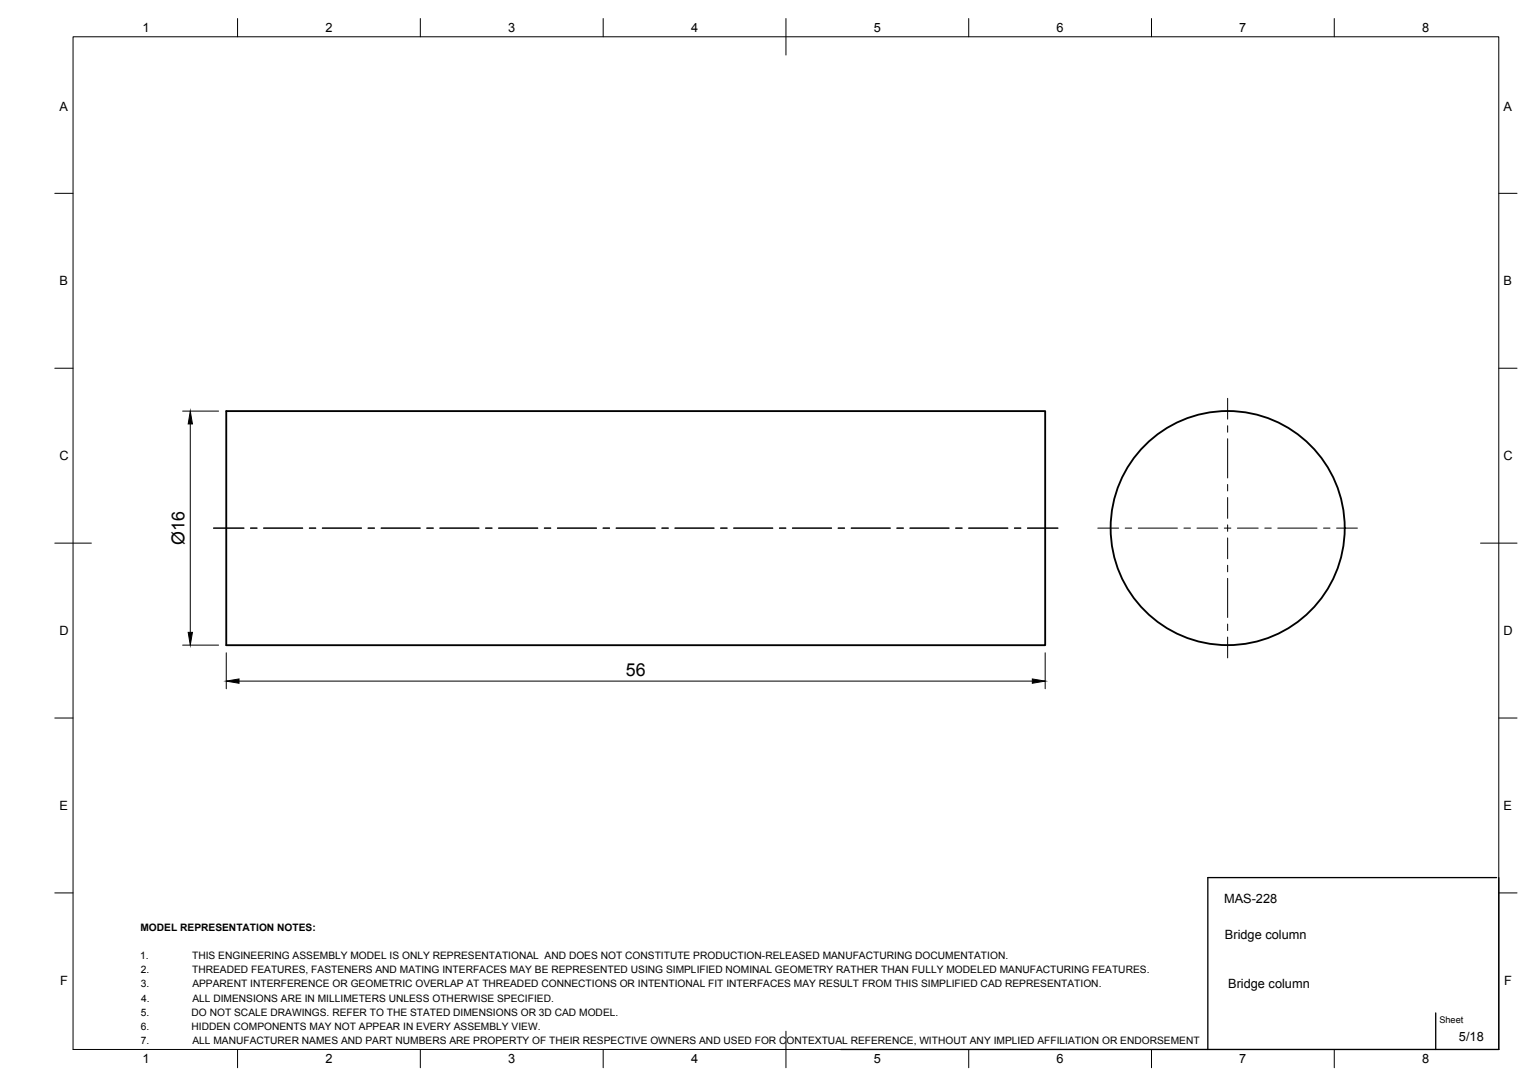
ISO-10303-21;
HEADER;
/* Generated by software containing ST-Developer
 * from STEP Tools, Inc. (www.steptools.com) 
 */

FILE_DESCRIPTION(
/* description */ ('Independent Peaucellier-Lipkin straight-line linkage. Radius arms 100
 mm, inversion-cell links 60 mm, crank radius and fixed-pivot spacing 
32 mm. Inversion constant 6400 mm squared, nominal output straight lin
e X=100 mm. Overhead bearing bridge clears the layered moving links. N
o accuracy or load rating assigned.'),
/* implementation_level */ '2;1');

FILE_NAME(
/* name */ 'Bridge column.step',
/* time_stamp */ '2026-11-09T18:06:16-08:00',
/* author */ (''),
/* organization */ (''),
/* preprocessor_version */ 'ST-DEVELOPER v20.2',
/* originating_system */ 'Autodesk Translation Framework v15.17.0.0',
/* authorisation */ '');

FILE_SCHEMA (('AUTOMOTIVE_DESIGN { 1 0 10303 214 3 1 1 }'));
ENDSEC;

DATA;
#10=MECHANICAL_DESIGN_GEOMETRIC_PRESENTATION_REPRESENTATION('',(#286),#3581);
#252=SHAPE_REPRESENTATION_RELATIONSHIP('SRR','None',#3686,#269);
#269=ADVANCED_BREP_SHAPE_REPRESENTATION('',(#303),#3568);
#286=STYLED_ITEM('',(#3777),#303);
#303=MANIFOLD_SOLID_BREP('Body1',#1872);
#382=PLANE('',#2136);
#383=PLANE('',#2137);
#455=FACE_OUTER_BOUND('',#584,.T.);
#456=FACE_OUTER_BOUND('',#585,.T.);
#457=FACE_OUTER_BOUND('',#586,.T.);
#584=EDGE_LOOP('',(#1448,#1449,#1450,#1451));
#585=EDGE_LOOP('',(#1452));
#586=EDGE_LOOP('',(#1453));
#737=LINE('',#3179,#835);
#835=VECTOR('',#2525,8.);
#915=CIRCLE('',#2134,8.);
#916=CIRCLE('',#2135,8.);
#1033=VERTEX_POINT('',#3176);
#1034=VERTEX_POINT('',#3178);
#1186=EDGE_CURVE('',#1033,#1033,#915,.T.);
#1187=EDGE_CURVE('',#1033,#1034,#737,.T.);
#1188=EDGE_CURVE('',#1034,#1034,#916,.T.);
#1448=ORIENTED_EDGE('',*,*,#1186,.F.);
#1449=ORIENTED_EDGE('',*,*,#1187,.T.);
#1450=ORIENTED_EDGE('',*,*,#1188,.T.);
#1451=ORIENTED_EDGE('',*,*,#1187,.F.);
#1452=ORIENTED_EDGE('',*,*,#1186,.T.);
#1453=ORIENTED_EDGE('',*,*,#1188,.F.);
#1720=CYLINDRICAL_SURFACE('',#2133,8.);
#1787=ADVANCED_FACE('',(#455),#1720,.T.);
#1788=ADVANCED_FACE('',(#456),#382,.T.);
#1789=ADVANCED_FACE('',(#457),#383,.F.);
#1872=CLOSED_SHELL('',(#1787,#1788,#1789));
#2132=AXIS2_PLACEMENT_3D('',#3174,#2519,#2520);
#2133=AXIS2_PLACEMENT_3D('',#3175,#2521,#2522);
#2134=AXIS2_PLACEMENT_3D('',#3177,#2523,#2524);
#2135=AXIS2_PLACEMENT_3D('',#3180,#2526,#2527);
#2136=AXIS2_PLACEMENT_3D('',#3181,#2528,#2529);
#2137=AXIS2_PLACEMENT_3D('',#3182,#2530,#2531);
#2519=DIRECTION('axis',(0.,0.,1.));
#2520=DIRECTION('refdir',(1.,0.,0.));
#2521=DIRECTION('center_axis',(0.,0.,1.));
#2522=DIRECTION('ref_axis',(1.,0.,0.));
#2523=DIRECTION('center_axis',(0.,0.,1.));
#2524=DIRECTION('ref_axis',(1.,0.,0.));
#2525=DIRECTION('',(0.,0.,-1.));
#2526=DIRECTION('center_axis',(0.,0.,1.));
#2527=DIRECTION('ref_axis',(1.,0.,0.));
#2528=DIRECTION('center_axis',(0.,0.,1.));
#2529=DIRECTION('ref_axis',(1.,0.,0.));
#2530=DIRECTION('center_axis',(0.,0.,1.));
#2531=DIRECTION('ref_axis',(1.,0.,0.));
#3174=CARTESIAN_POINT('',(0.,0.,0.));
#3175=CARTESIAN_POINT('Origin',(0.,0.,0.));
#3176=CARTESIAN_POINT('',(-8.,-9.79717439317883E-16,56.));
#3177=CARTESIAN_POINT('Origin',(0.,0.,56.));
#3178=CARTESIAN_POINT('',(-8.,-9.79717439317883E-16,0.));
#3179=CARTESIAN_POINT('',(-8.,-9.79717439317883E-16,0.));
#3180=CARTESIAN_POINT('Origin',(0.,0.,0.));
#3181=CARTESIAN_POINT('Origin',(0.,0.,56.));
#3182=CARTESIAN_POINT('Origin',(0.,0.,0.));
#3549=UNCERTAINTY_MEASURE_WITH_UNIT(LENGTH_MEASURE(0.01),#3582,
'DISTANCE_ACCURACY_VALUE',
'Maximum model space distance between geometric entities at asserted c
onnectivities');
#3562=UNCERTAINTY_MEASURE_WITH_UNIT(LENGTH_MEASURE(0.01),#3582,
'DISTANCE_ACCURACY_VALUE',
'Maximum model space distance between geometric entities at asserted c
onnectivities');
#3568=(
GEOMETRIC_REPRESENTATION_CONTEXT(3)
GLOBAL_UNCERTAINTY_ASSIGNED_CONTEXT((#3549))
GLOBAL_UNIT_ASSIGNED_CONTEXT((#3582,#3584,#3585))
REPRESENTATION_CONTEXT('','3D')
);
#3581=(
GEOMETRIC_REPRESENTATION_CONTEXT(3)
GLOBAL_UNCERTAINTY_ASSIGNED_CONTEXT((#3562))
GLOBAL_UNIT_ASSIGNED_CONTEXT((#3582,#3584,#3585))
REPRESENTATION_CONTEXT('','3D')
);
#3582=(
LENGTH_UNIT()
NAMED_UNIT(*)
SI_UNIT(.MILLI.,.METRE.)
);
#3584=(
NAMED_UNIT(*)
PLANE_ANGLE_UNIT()
SI_UNIT($,.RADIAN.)
);
#3585=(
NAMED_UNIT(*)
SI_UNIT($,.STERADIAN.)
SOLID_ANGLE_UNIT()
);
#3591=SHAPE_DEFINITION_REPRESENTATION(#3609,#3686);
#3609=PRODUCT_DEFINITION_SHAPE('',$,#3705);
#3686=SHAPE_REPRESENTATION('',(#2132),#3568);
#3699=PRODUCT_DEFINITION_CONTEXT('part definition',#3755,'design');
#3705=PRODUCT_DEFINITION('Bridge column','Bridge column',#3723,#3699);
#3723=PRODUCT_DEFINITION_FORMATION('',$,#3762);
#3755=APPLICATION_CONTEXT(
'Core Data for Automotive Mechanical Design Process');
#3756=PRODUCT_CONTEXT('part definition',#3755,'mechanical');
#3762=PRODUCT('Bridge column','Bridge column',$,(#3756));
#3777=PRESENTATION_STYLE_ASSIGNMENT((#3790));
#3790=SURFACE_STYLE_USAGE(.BOTH.,#3803);
#3803=SURFACE_SIDE_STYLE('',(#3816));
#3816=SURFACE_STYLE_FILL_AREA(#3829);
#3829=FILL_AREA_STYLE('Support gray',(#3842));
#3842=FILL_AREA_STYLE_COLOUR('Support gray',#3855);
#3855=COLOUR_RGB('Support gray',0.407843137254902,0.447058823529412,0.498039215686275);
ENDSEC;
END-ISO-10303-21;
